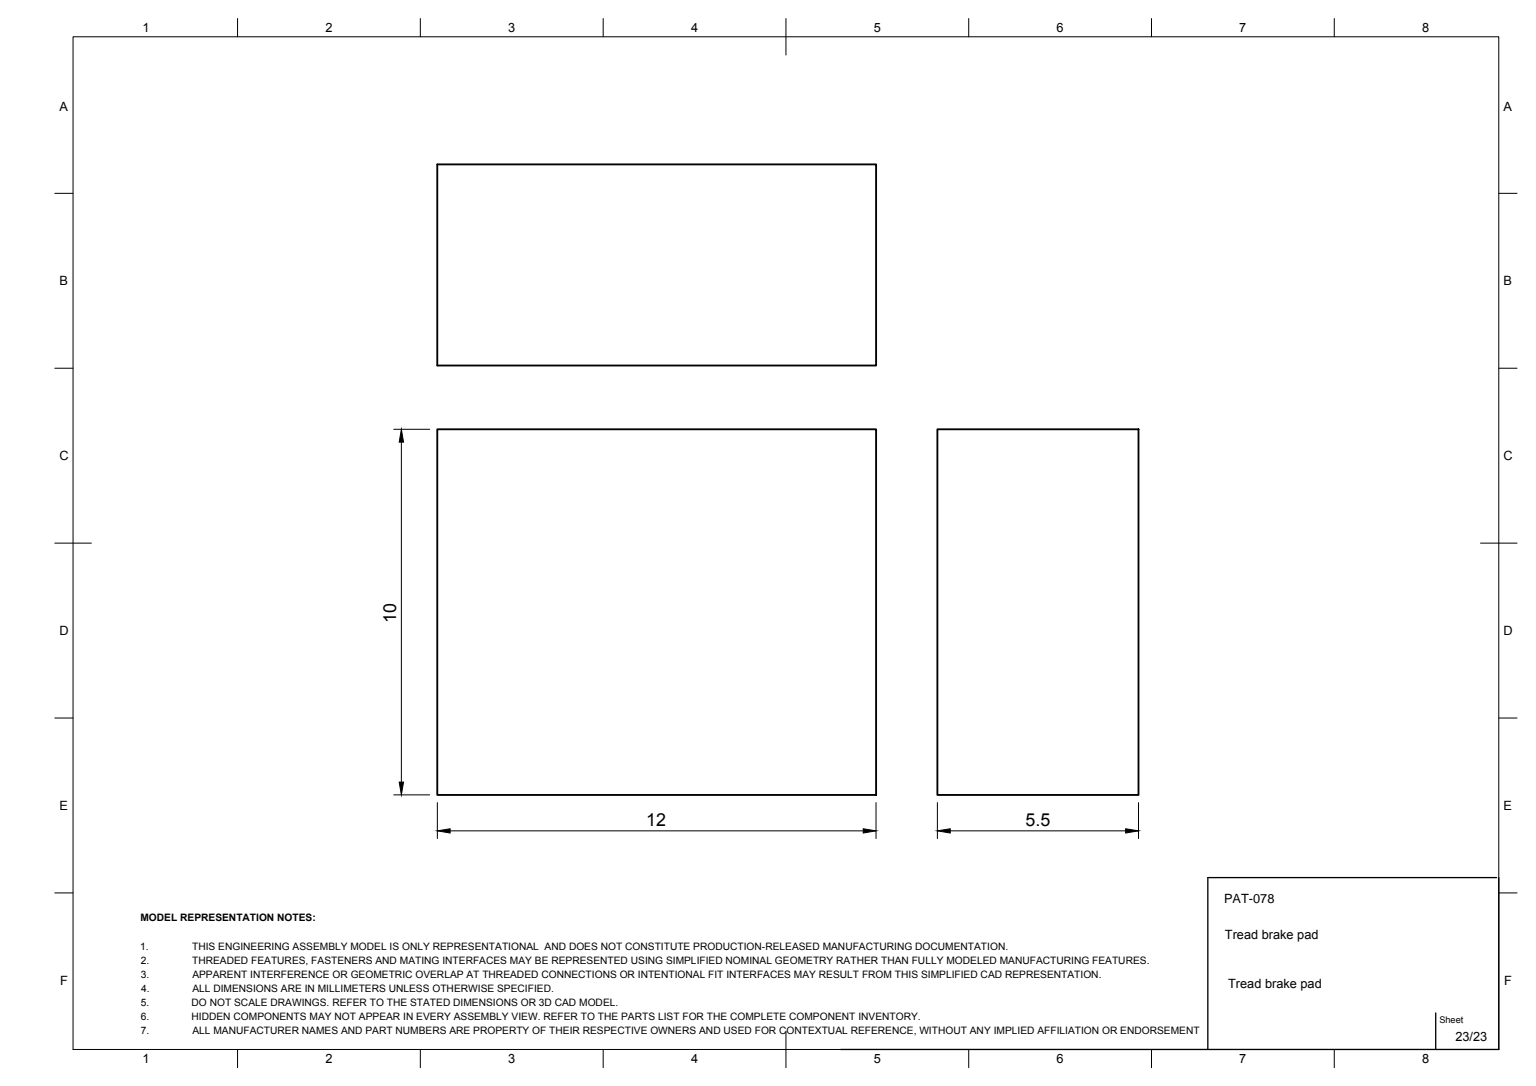
ISO-10303-21;
HEADER;
/* Generated by software containing ST-Developer
 * from STEP Tools, Inc. (www.steptools.com) 
 */

FILE_DESCRIPTION(
/* description */ ('Pedal-braked fixed caster'),
/* implementation_level */ '2;1');

FILE_NAME(
/* name */ 'Tread brake pad.step',
/* time_stamp */ '2026-10-28T03:26:52-07:00',
/* author */ (''),
/* organization */ (''),
/* preprocessor_version */ 'ST-DEVELOPER v20.2',
/* originating_system */ 'Autodesk Translation Framework v15.17.0.0',
/* authorisation */ '');

FILE_SCHEMA (('AUTOMOTIVE_DESIGN { 1 0 10303 214 3 1 1 }'));
ENDSEC;

DATA;
#10=MECHANICAL_DESIGN_GEOMETRIC_PRESENTATION_REPRESENTATION('',(#229),#5734);
#188=SHAPE_REPRESENTATION_RELATIONSHIP('SRR','None',#5829,#205);
#205=ADVANCED_BREP_SHAPE_REPRESENTATION('',(#252),#5733);
#229=STYLED_ITEM('',(#5970),#252);
#252=MANIFOLD_SOLID_BREP('Body1',#3011);
#648=FACE_OUTER_BOUND('',#871,.T.);
#649=FACE_OUTER_BOUND('',#872,.T.);
#650=FACE_OUTER_BOUND('',#873,.T.);
#651=FACE_OUTER_BOUND('',#874,.T.);
#652=FACE_OUTER_BOUND('',#875,.T.);
#653=FACE_OUTER_BOUND('',#876,.T.);
#871=EDGE_LOOP('',(#2676,#2677,#2678,#2679));
#872=EDGE_LOOP('',(#2680,#2681,#2682,#2683));
#873=EDGE_LOOP('',(#2684,#2685,#2686,#2687));
#874=EDGE_LOOP('',(#2688,#2689,#2690,#2691));
#875=EDGE_LOOP('',(#2692,#2693,#2694,#2695));
#876=EDGE_LOOP('',(#2696,#2697,#2698,#2699));
#1077=LINE('',#5661,#1289);
#1078=LINE('',#5663,#1290);
#1079=LINE('',#5665,#1291);
#1080=LINE('',#5666,#1292);
#1081=LINE('',#5669,#1293);
#1082=LINE('',#5671,#1294);
#1083=LINE('',#5672,#1295);
#1084=LINE('',#5675,#1296);
#1085=LINE('',#5677,#1297);
#1086=LINE('',#5678,#1298);
#1087=LINE('',#5680,#1299);
#1088=LINE('',#5681,#1300);
#1289=VECTOR('',#4463,1.);
#1290=VECTOR('',#4464,1.);
#1291=VECTOR('',#4465,1.);
#1292=VECTOR('',#4466,1.);
#1293=VECTOR('',#4469,1.);
#1294=VECTOR('',#4470,1.);
#1295=VECTOR('',#4471,1.);
#1296=VECTOR('',#4474,1.);
#1297=VECTOR('',#4475,1.);
#1298=VECTOR('',#4476,1.);
#1299=VECTOR('',#4479,1.);
#1300=VECTOR('',#4480,1.);
#1552=VERTEX_POINT('',#5659);
#1553=VERTEX_POINT('',#5660);
#1554=VERTEX_POINT('',#5662);
#1555=VERTEX_POINT('',#5664);
#1556=VERTEX_POINT('',#5668);
#1557=VERTEX_POINT('',#5670);
#1558=VERTEX_POINT('',#5674);
#1559=VERTEX_POINT('',#5676);
#1928=EDGE_CURVE('',#1552,#1553,#1077,.T.);
#1929=EDGE_CURVE('',#1553,#1554,#1078,.T.);
#1930=EDGE_CURVE('',#1555,#1554,#1079,.T.);
#1931=EDGE_CURVE('',#1552,#1555,#1080,.T.);
#1932=EDGE_CURVE('',#1556,#1552,#1081,.T.);
#1933=EDGE_CURVE('',#1557,#1555,#1082,.T.);
#1934=EDGE_CURVE('',#1556,#1557,#1083,.T.);
#1935=EDGE_CURVE('',#1558,#1556,#1084,.T.);
#1936=EDGE_CURVE('',#1559,#1557,#1085,.T.);
#1937=EDGE_CURVE('',#1558,#1559,#1086,.T.);
#1938=EDGE_CURVE('',#1553,#1558,#1087,.T.);
#1939=EDGE_CURVE('',#1554,#1559,#1088,.T.);
#2676=ORIENTED_EDGE('',*,*,#1928,.T.);
#2677=ORIENTED_EDGE('',*,*,#1929,.T.);
#2678=ORIENTED_EDGE('',*,*,#1930,.F.);
#2679=ORIENTED_EDGE('',*,*,#1931,.F.);
#2680=ORIENTED_EDGE('',*,*,#1932,.T.);
#2681=ORIENTED_EDGE('',*,*,#1931,.T.);
#2682=ORIENTED_EDGE('',*,*,#1933,.F.);
#2683=ORIENTED_EDGE('',*,*,#1934,.F.);
#2684=ORIENTED_EDGE('',*,*,#1935,.T.);
#2685=ORIENTED_EDGE('',*,*,#1934,.T.);
#2686=ORIENTED_EDGE('',*,*,#1936,.F.);
#2687=ORIENTED_EDGE('',*,*,#1937,.F.);
#2688=ORIENTED_EDGE('',*,*,#1938,.T.);
#2689=ORIENTED_EDGE('',*,*,#1937,.T.);
#2690=ORIENTED_EDGE('',*,*,#1939,.F.);
#2691=ORIENTED_EDGE('',*,*,#1929,.F.);
#2692=ORIENTED_EDGE('',*,*,#1939,.T.);
#2693=ORIENTED_EDGE('',*,*,#1936,.T.);
#2694=ORIENTED_EDGE('',*,*,#1933,.T.);
#2695=ORIENTED_EDGE('',*,*,#1930,.T.);
#2696=ORIENTED_EDGE('',*,*,#1938,.F.);
#2697=ORIENTED_EDGE('',*,*,#1928,.F.);
#2698=ORIENTED_EDGE('',*,*,#1932,.F.);
#2699=ORIENTED_EDGE('',*,*,#1935,.F.);
#2803=PLANE('',#3550);
#2804=PLANE('',#3551);
#2805=PLANE('',#3552);
#2806=PLANE('',#3553);
#2807=PLANE('',#3554);
#2808=PLANE('',#3555);
#2981=ADVANCED_FACE('',(#648),#2803,.T.);
#2982=ADVANCED_FACE('',(#649),#2804,.T.);
#2983=ADVANCED_FACE('',(#650),#2805,.T.);
#2984=ADVANCED_FACE('',(#651),#2806,.T.);
#2985=ADVANCED_FACE('',(#652),#2807,.T.);
#2986=ADVANCED_FACE('',(#653),#2808,.F.);
#3011=CLOSED_SHELL('',(#2981,#2982,#2983,#2984,#2985,#2986));
#3549=AXIS2_PLACEMENT_3D('',#5657,#4459,#4460);
#3550=AXIS2_PLACEMENT_3D('',#5658,#4461,#4462);
#3551=AXIS2_PLACEMENT_3D('',#5667,#4467,#4468);
#3552=AXIS2_PLACEMENT_3D('',#5673,#4472,#4473);
#3553=AXIS2_PLACEMENT_3D('',#5679,#4477,#4478);
#3554=AXIS2_PLACEMENT_3D('',#5682,#4481,#4482);
#3555=AXIS2_PLACEMENT_3D('',#5683,#4483,#4484);
#4459=DIRECTION('axis',(0.,0.,1.));
#4460=DIRECTION('refdir',(1.,0.,0.));
#4461=DIRECTION('center_axis',(0.,1.,0.));
#4462=DIRECTION('ref_axis',(-1.,0.,0.));
#4463=DIRECTION('',(-1.,0.,0.));
#4464=DIRECTION('',(0.,0.,1.));
#4465=DIRECTION('',(-1.,0.,0.));
#4466=DIRECTION('',(0.,0.,1.));
#4467=DIRECTION('center_axis',(1.,0.,0.));
#4468=DIRECTION('ref_axis',(0.,1.,0.));
#4469=DIRECTION('',(0.,1.,0.));
#4470=DIRECTION('',(0.,1.,0.));
#4471=DIRECTION('',(0.,0.,1.));
#4472=DIRECTION('center_axis',(0.,-1.,0.));
#4473=DIRECTION('ref_axis',(1.,0.,0.));
#4474=DIRECTION('',(1.,0.,0.));
#4475=DIRECTION('',(1.,0.,0.));
#4476=DIRECTION('',(0.,0.,1.));
#4477=DIRECTION('center_axis',(-1.,0.,0.));
#4478=DIRECTION('ref_axis',(0.,-1.,0.));
#4479=DIRECTION('',(0.,-1.,0.));
#4480=DIRECTION('',(0.,-1.,0.));
#4481=DIRECTION('center_axis',(0.,0.,1.));
#4482=DIRECTION('ref_axis',(1.,0.,0.));
#4483=DIRECTION('center_axis',(0.,0.,1.));
#4484=DIRECTION('ref_axis',(1.,0.,0.));
#5657=CARTESIAN_POINT('',(0.,0.,0.));
#5658=CARTESIAN_POINT('Origin',(0.5,0.6,8.75));
#5659=CARTESIAN_POINT('',(0.5,0.6,8.75));
#5660=CARTESIAN_POINT('',(-0.5,0.6,8.75));
#5661=CARTESIAN_POINT('',(0.5,0.6,8.75));
#5662=CARTESIAN_POINT('',(-0.5,0.6,9.3));
#5663=CARTESIAN_POINT('',(-0.5,0.6,8.75));
#5664=CARTESIAN_POINT('',(0.5,0.6,9.3));
#5665=CARTESIAN_POINT('',(0.5,0.6,9.3));
#5666=CARTESIAN_POINT('',(0.5,0.6,8.75));
#5667=CARTESIAN_POINT('Origin',(0.5,-0.6,8.75));
#5668=CARTESIAN_POINT('',(0.5,-0.6,8.75));
#5669=CARTESIAN_POINT('',(0.5,-0.6,8.75));
#5670=CARTESIAN_POINT('',(0.5,-0.6,9.3));
#5671=CARTESIAN_POINT('',(0.5,-0.6,9.3));
#5672=CARTESIAN_POINT('',(0.5,-0.6,8.75));
#5673=CARTESIAN_POINT('Origin',(-0.5,-0.6,8.75));
#5674=CARTESIAN_POINT('',(-0.5,-0.6,8.75));
#5675=CARTESIAN_POINT('',(-0.5,-0.6,8.75));
#5676=CARTESIAN_POINT('',(-0.5,-0.6,9.3));
#5677=CARTESIAN_POINT('',(-0.5,-0.6,9.3));
#5678=CARTESIAN_POINT('',(-0.5,-0.6,8.75));
#5679=CARTESIAN_POINT('Origin',(-0.5,0.6,8.75));
#5680=CARTESIAN_POINT('',(-0.5,0.6,8.75));
#5681=CARTESIAN_POINT('',(-0.5,0.6,9.3));
#5682=CARTESIAN_POINT('Origin',(0.,0.,9.3));
#5683=CARTESIAN_POINT('Origin',(0.,0.,8.75));
#5710=UNCERTAINTY_MEASURE_WITH_UNIT(LENGTH_MEASURE(0.001),#5735,
'DISTANCE_ACCURACY_VALUE',
'Maximum model space distance between geometric entities at asserted c
onnectivities');
#5711=UNCERTAINTY_MEASURE_WITH_UNIT(LENGTH_MEASURE(0.001),#5735,
'DISTANCE_ACCURACY_VALUE',
'Maximum model space distance between geometric entities at asserted c
onnectivities');
#5733=(
GEOMETRIC_REPRESENTATION_CONTEXT(3)
GLOBAL_UNCERTAINTY_ASSIGNED_CONTEXT((#5710))
GLOBAL_UNIT_ASSIGNED_CONTEXT((#5735,#5737,#5738))
REPRESENTATION_CONTEXT('','3D')
);
#5734=(
GEOMETRIC_REPRESENTATION_CONTEXT(3)
GLOBAL_UNCERTAINTY_ASSIGNED_CONTEXT((#5711))
GLOBAL_UNIT_ASSIGNED_CONTEXT((#5735,#5737,#5738))
REPRESENTATION_CONTEXT('','3D')
);
#5735=(
LENGTH_UNIT()
NAMED_UNIT(*)
SI_UNIT(.CENTI.,.METRE.)
);
#5737=(
NAMED_UNIT(*)
PLANE_ANGLE_UNIT()
SI_UNIT($,.RADIAN.)
);
#5738=(
NAMED_UNIT(*)
SI_UNIT($,.STERADIAN.)
SOLID_ANGLE_UNIT()
);
#5760=SHAPE_DEFINITION_REPRESENTATION(#5802,#5829);
#5802=PRODUCT_DEFINITION_SHAPE('',$,#5852);
#5829=SHAPE_REPRESENTATION('',(#3549),#5733);
#5830=PRODUCT_DEFINITION_CONTEXT('part definition',#5898,'design');
#5852=PRODUCT_DEFINITION('Tread brake pad','Tread brake pad',#5874,#5830);
#5874=PRODUCT_DEFINITION_FORMATION('',$,#5921);
#5898=APPLICATION_CONTEXT(
'Core Data for Automotive Mechanical Design Process');
#5899=PRODUCT_CONTEXT('part definition',#5898,'mechanical');
#5921=PRODUCT('Tread brake pad','Tread brake pad','Tread brake pad',(#5899));
#5964=COLOUR_RGB('Light Blue',0.38,0.62,0.78);
#5965=FILL_AREA_STYLE_COLOUR('',#5964);
#5966=FILL_AREA_STYLE('',(#5965));
#5967=SURFACE_STYLE_FILL_AREA(#5966);
#5968=SURFACE_SIDE_STYLE('',(#5967));
#5969=SURFACE_STYLE_USAGE(.BOTH.,#5968);
#5970=PRESENTATION_STYLE_ASSIGNMENT((#5969));
ENDSEC;
END-ISO-10303-21;
